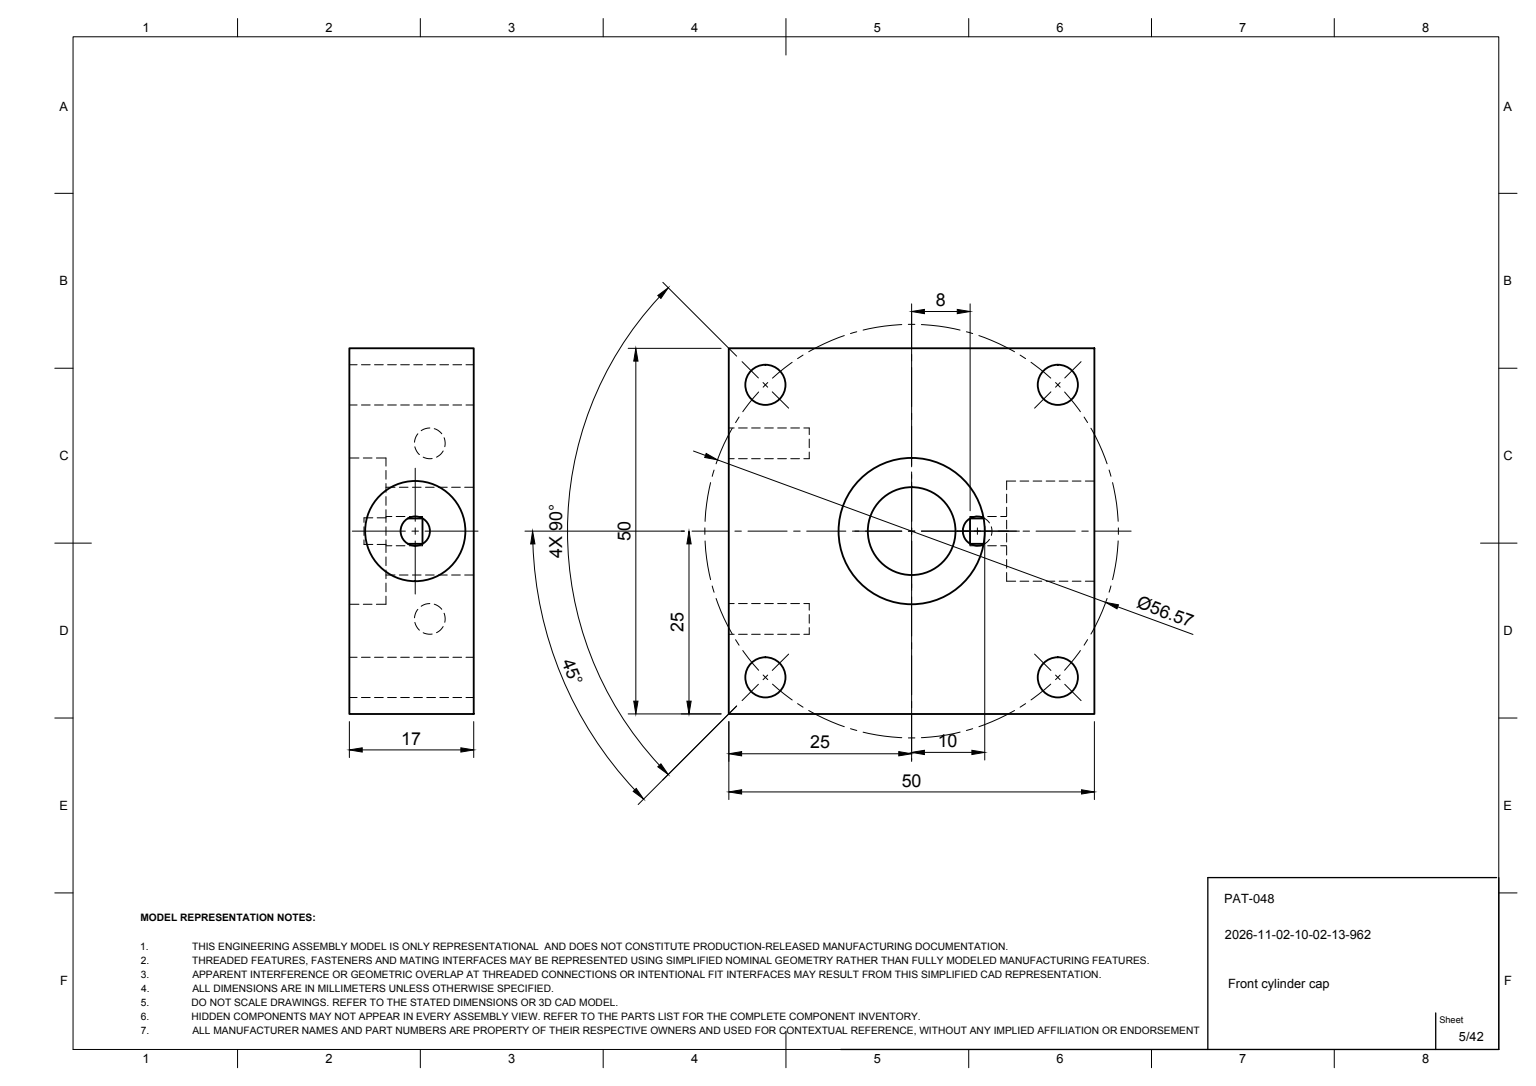
ISO-10303-21;
HEADER;
/* Generated by software containing ST-Developer
 * from STEP Tools, Inc. (www.steptools.com) 
 */

FILE_DESCRIPTION(
/* description */ ('Guided pneumatic stop gate'),
/* implementation_level */ '2;1');

FILE_NAME(
/* name */ 'Front cylinder cap.step',
/* time_stamp */ '2026-10-27T21:43:45-07:00',
/* author */ (''),
/* organization */ (''),
/* preprocessor_version */ 'ST-DEVELOPER v20.2',
/* originating_system */ 'Autodesk Translation Framework v15.17.0.0',
/* authorisation */ '');

FILE_SCHEMA (('AUTOMOTIVE_DESIGN { 1 0 10303 214 3 1 1 }'));
ENDSEC;

DATA;
#10=MECHANICAL_DESIGN_GEOMETRIC_PRESENTATION_REPRESENTATION('',(#535),#14392);
#451=SHAPE_REPRESENTATION_RELATIONSHIP('SRR','None',#14585,#493);
#493=ADVANCED_BREP_SHAPE_REPRESENTATION('',(#577),#14347);
#535=STYLED_ITEM('',(#14877),#577);
#577=MANIFOLD_SOLID_BREP('Body1',#7875);
#615=FACE_BOUND('',#1613,.T.);
#616=FACE_BOUND('',#1620,.T.);
#617=FACE_BOUND('',#1622,.T.);
#618=FACE_BOUND('',#1623,.T.);
#619=FACE_BOUND('',#1624,.T.);
#620=FACE_BOUND('',#1625,.T.);
#621=FACE_BOUND('',#1626,.T.);
#622=FACE_BOUND('',#1629,.T.);
#623=FACE_BOUND('',#1630,.T.);
#624=FACE_BOUND('',#1631,.T.);
#625=FACE_BOUND('',#1632,.T.);
#626=FACE_BOUND('',#1633,.T.);
#627=FACE_BOUND('',#1636,.T.);
#628=FACE_BOUND('',#1638,.T.);
#629=FACE_BOUND('',#1639,.T.);
#825=ELLIPSE('',#8400,0.282842712474619,0.2);
#826=ELLIPSE('',#8401,0.282842712474619,0.2);
#827=ELLIPSE('',#8403,0.282842712474619,0.2);
#828=ELLIPSE('',#8404,0.282842712474619,0.2);
#829=ELLIPSE('',#8408,0.282842712474619,0.2);
#830=ELLIPSE('',#8410,0.282842712474619,0.2);
#831=ELLIPSE('',#8412,0.282842712474619,0.2);
#839=PLANE('',#8390);
#840=PLANE('',#8394);
#841=PLANE('',#8395);
#842=PLANE('',#8397);
#843=PLANE('',#8413);
#844=PLANE('',#8415);
#845=PLANE('',#8416);
#846=PLANE('',#8418);
#847=PLANE('',#8429);
#848=PLANE('',#8433);
#849=PLANE('',#8449);
#850=PLANE('',#8450);
#851=PLANE('',#8451);
#852=PLANE('',#8452);
#853=PLANE('',#8453);
#854=PLANE('',#8454);
#855=PLANE('',#8455);
#1118=FACE_OUTER_BOUND('',#1593,.T.);
#1119=FACE_OUTER_BOUND('',#1594,.T.);
#1120=FACE_OUTER_BOUND('',#1595,.T.);
#1121=FACE_OUTER_BOUND('',#1596,.T.);
#1122=FACE_OUTER_BOUND('',#1597,.T.);
#1123=FACE_OUTER_BOUND('',#1598,.T.);
#1124=FACE_OUTER_BOUND('',#1599,.T.);
#1125=FACE_OUTER_BOUND('',#1600,.T.);
#1126=FACE_OUTER_BOUND('',#1601,.T.);
#1127=FACE_OUTER_BOUND('',#1602,.T.);
#1128=FACE_OUTER_BOUND('',#1603,.T.);
#1129=FACE_OUTER_BOUND('',#1604,.T.);
#1130=FACE_OUTER_BOUND('',#1605,.T.);
#1131=FACE_OUTER_BOUND('',#1606,.T.);
#1132=FACE_OUTER_BOUND('',#1607,.T.);
#1133=FACE_OUTER_BOUND('',#1608,.T.);
#1134=FACE_OUTER_BOUND('',#1609,.T.);
#1135=FACE_OUTER_BOUND('',#1610,.T.);
#1136=FACE_OUTER_BOUND('',#1611,.T.);
#1137=FACE_OUTER_BOUND('',#1612,.T.);
#1138=FACE_OUTER_BOUND('',#1614,.T.);
#1139=FACE_OUTER_BOUND('',#1615,.T.);
#1140=FACE_OUTER_BOUND('',#1616,.T.);
#1141=FACE_OUTER_BOUND('',#1617,.T.);
#1142=FACE_OUTER_BOUND('',#1618,.T.);
#1143=FACE_OUTER_BOUND('',#1619,.T.);
#1144=FACE_OUTER_BOUND('',#1621,.T.);
#1145=FACE_OUTER_BOUND('',#1627,.T.);
#1146=FACE_OUTER_BOUND('',#1628,.T.);
#1147=FACE_OUTER_BOUND('',#1634,.T.);
#1148=FACE_OUTER_BOUND('',#1635,.T.);
#1149=FACE_OUTER_BOUND('',#1637,.T.);
#1593=EDGE_LOOP('',(#5316,#5317,#5318,#5319));
#1594=EDGE_LOOP('',(#5320));
#1595=EDGE_LOOP('',(#5321,#5322,#5323,#5324));
#1596=EDGE_LOOP('',(#5325));
#1597=EDGE_LOOP('',(#5326,#5327));
#1598=EDGE_LOOP('',(#5328,#5329));
#1599=EDGE_LOOP('',(#5330,#5331,#5332));
#1600=EDGE_LOOP('',(#5333,#5334,#5335,#5336,#5337,#5338,#5339,#5340,#5341,
#5342,#5343,#5344,#5345));
#1601=EDGE_LOOP('',(#5346,#5347,#5348));
#1602=EDGE_LOOP('',(#5349,#5350));
#1603=EDGE_LOOP('',(#5351,#5352));
#1604=EDGE_LOOP('',(#5353,#5354));
#1605=EDGE_LOOP('',(#5355,#5356));
#1606=EDGE_LOOP('',(#5357,#5358,#5359));
#1607=EDGE_LOOP('',(#5360,#5361,#5362,#5363,#5364,#5365,#5366,#5367,#5368));
#1608=EDGE_LOOP('',(#5369,#5370,#5371));
#1609=EDGE_LOOP('',(#5372,#5373,#5374,#5375,#5376,#5377,#5378,#5379));
#1610=EDGE_LOOP('',(#5380,#5381));
#1611=EDGE_LOOP('',(#5382,#5383,#5384,#5385));
#1612=EDGE_LOOP('',(#5386));
#1613=EDGE_LOOP('',(#5387));
#1614=EDGE_LOOP('',(#5388,#5389,#5390,#5391));
#1615=EDGE_LOOP('',(#5392,#5393,#5394,#5395));
#1616=EDGE_LOOP('',(#5396,#5397,#5398,#5399));
#1617=EDGE_LOOP('',(#5400,#5401,#5402,#5403));
#1618=EDGE_LOOP('',(#5404,#5405,#5406,#5407));
#1619=EDGE_LOOP('',(#5408,#5409,#5410,#5411));
#1620=EDGE_LOOP('',(#5412));
#1621=EDGE_LOOP('',(#5413,#5414,#5415,#5416));
#1622=EDGE_LOOP('',(#5417));
#1623=EDGE_LOOP('',(#5418));
#1624=EDGE_LOOP('',(#5419));
#1625=EDGE_LOOP('',(#5420));
#1626=EDGE_LOOP('',(#5421));
#1627=EDGE_LOOP('',(#5422,#5423,#5424,#5425));
#1628=EDGE_LOOP('',(#5426,#5427,#5428,#5429));
#1629=EDGE_LOOP('',(#5430));
#1630=EDGE_LOOP('',(#5431));
#1631=EDGE_LOOP('',(#5432));
#1632=EDGE_LOOP('',(#5433));
#1633=EDGE_LOOP('',(#5434));
#1634=EDGE_LOOP('',(#5435,#5436,#5437,#5438));
#1635=EDGE_LOOP('',(#5439,#5440,#5441,#5442));
#1636=EDGE_LOOP('',(#5443));
#1637=EDGE_LOOP('',(#5444,#5445,#5446,#5447));
#1638=EDGE_LOOP('',(#5448));
#1639=EDGE_LOOP('',(#5449));
#2278=LINE('',#11927,#2823);
#2279=LINE('',#11934,#2824);
#2280=LINE('',#11940,#2825);
#2281=LINE('',#11944,#2826);
#2282=LINE('',#11952,#2827);
#2283=LINE('',#11954,#2828);
#2284=LINE('',#11959,#2829);
#2285=LINE('',#11963,#2830);
#2286=LINE('',#11967,#2831);
#2287=LINE('',#11978,#2832);
#2288=LINE('',#11986,#2833);
#2289=LINE('',#11994,#2834);
#2290=LINE('',#12002,#2835);
#2291=LINE('',#12009,#2836);
#2292=LINE('',#12015,#2837);
#2293=LINE('',#12021,#2838);
#2294=LINE('',#12027,#2839);
#2295=LINE('',#12033,#2840);
#2296=LINE('',#12039,#2841);
#2297=LINE('',#12041,#2842);
#2298=LINE('',#12043,#2843);
#2299=LINE('',#12044,#2844);
#2300=LINE('',#12047,#2845);
#2301=LINE('',#12049,#2846);
#2302=LINE('',#12050,#2847);
#2303=LINE('',#12053,#2848);
#2304=LINE('',#12055,#2849);
#2305=LINE('',#12056,#2850);
#2306=LINE('',#12058,#2851);
#2307=LINE('',#12059,#2852);
#2823=VECTOR('',#9391,0.21);
#2824=VECTOR('',#9400,0.21);
#2825=VECTOR('',#9407,1.);
#2826=VECTOR('',#9412,1.);
#2827=VECTOR('',#9423,1.);
#2828=VECTOR('',#9424,1.);
#2829=VECTOR('',#9429,0.2);
#2830=VECTOR('',#9432,1.);
#2831=VECTOR('',#9435,1.);
#2832=VECTOR('',#9454,1.);
#2833=VECTOR('',#9467,0.2);
#2834=VECTOR('',#9478,1.);
#2835=VECTOR('',#9489,0.685);
#2836=VECTOR('',#9498,0.275);
#2837=VECTOR('',#9505,0.275);
#2838=VECTOR('',#9512,0.275);
#2839=VECTOR('',#9519,0.275);
#2840=VECTOR('',#9526,0.6);
#2841=VECTOR('',#9533,1.);
#2842=VECTOR('',#9534,1.);
#2843=VECTOR('',#9535,1.);
#2844=VECTOR('',#9536,1.);
#2845=VECTOR('',#9539,1.);
#2846=VECTOR('',#9540,1.);
#2847=VECTOR('',#9541,1.);
#2848=VECTOR('',#9544,1.);
#2849=VECTOR('',#9545,1.);
#2850=VECTOR('',#9546,1.);
#2851=VECTOR('',#9549,1.);
#2852=VECTOR('',#9550,1.);
#3368=CIRCLE('',#8388,0.21);
#3369=CIRCLE('',#8389,0.21);
#3370=CIRCLE('',#8392,0.21);
#3371=CIRCLE('',#8393,0.21);
#3372=CIRCLE('',#8396,0.2);
#3373=CIRCLE('',#8398,0.2);
#3374=CIRCLE('',#8405,0.2);
#3375=CIRCLE('',#8406,0.2);
#3376=CIRCLE('',#8407,0.2);
#3377=CIRCLE('',#8411,0.2);
#3378=CIRCLE('',#8414,1.);
#3379=CIRCLE('',#8417,0.2);
#3380=CIRCLE('',#8419,0.2);
#3381=CIRCLE('',#8422,0.2);
#3382=CIRCLE('',#8424,0.2);
#3383=CIRCLE('',#8426,1.);
#3384=CIRCLE('',#8427,1.);
#3385=CIRCLE('',#8428,1.);
#3386=CIRCLE('',#8431,0.685);
#3387=CIRCLE('',#8432,0.685);
#3388=CIRCLE('',#8435,0.275);
#3389=CIRCLE('',#8436,0.275);
#3390=CIRCLE('',#8438,0.275);
#3391=CIRCLE('',#8439,0.275);
#3392=CIRCLE('',#8441,0.275);
#3393=CIRCLE('',#8442,0.275);
#3394=CIRCLE('',#8444,0.275);
#3395=CIRCLE('',#8445,0.275);
#3396=CIRCLE('',#8447,0.6);
#3397=CIRCLE('',#8448,0.6);
#3737=VERTEX_POINT('',#11924);
#3738=VERTEX_POINT('',#11926);
#3739=VERTEX_POINT('',#11931);
#3740=VERTEX_POINT('',#11933);
#3741=VERTEX_POINT('',#11938);
#3742=VERTEX_POINT('',#11939);
#3743=VERTEX_POINT('',#11943);
#3744=VERTEX_POINT('',#11947);
#3745=VERTEX_POINT('',#11951);
#3746=VERTEX_POINT('',#11953);
#3747=VERTEX_POINT('',#11956);
#3748=VERTEX_POINT('',#11958);
#3749=VERTEX_POINT('',#11960);
#3750=VERTEX_POINT('',#11962);
#3751=VERTEX_POINT('',#11964);
#3752=VERTEX_POINT('',#11966);
#3753=VERTEX_POINT('',#11971);
#3754=VERTEX_POINT('',#11985);
#3755=VERTEX_POINT('',#11991);
#3756=VERTEX_POINT('',#11993);
#3757=VERTEX_POINT('',#11999);
#3758=VERTEX_POINT('',#12001);
#3759=VERTEX_POINT('',#12006);
#3760=VERTEX_POINT('',#12008);
#3761=VERTEX_POINT('',#12012);
#3762=VERTEX_POINT('',#12014);
#3763=VERTEX_POINT('',#12018);
#3764=VERTEX_POINT('',#12020);
#3765=VERTEX_POINT('',#12024);
#3766=VERTEX_POINT('',#12026);
#3767=VERTEX_POINT('',#12030);
#3768=VERTEX_POINT('',#12032);
#3769=VERTEX_POINT('',#12037);
#3770=VERTEX_POINT('',#12038);
#3771=VERTEX_POINT('',#12040);
#3772=VERTEX_POINT('',#12042);
#3773=VERTEX_POINT('',#12046);
#3774=VERTEX_POINT('',#12048);
#3775=VERTEX_POINT('',#12052);
#3776=VERTEX_POINT('',#12054);
#4356=EDGE_CURVE('',#3737,#3737,#3368,.T.);
#4357=EDGE_CURVE('',#3737,#3738,#2278,.T.);
#4358=EDGE_CURVE('',#3738,#3738,#3369,.T.);
#4359=EDGE_CURVE('',#3739,#3739,#3370,.T.);
#4360=EDGE_CURVE('',#3739,#3740,#2279,.T.);
#4361=EDGE_CURVE('',#3740,#3740,#3371,.T.);
#4362=EDGE_CURVE('',#3741,#3742,#2280,.T.);
#4363=EDGE_CURVE('',#3741,#3742,#3372,.T.);
#4364=EDGE_CURVE('',#3743,#3741,#2281,.T.);
#4365=EDGE_CURVE('',#3743,#3741,#3373,.T.);
#4366=EDGE_CURVE('',#3744,#3743,#825,.T.);
#4367=EDGE_CURVE('',#3741,#3744,#826,.T.);
#4368=EDGE_CURVE('',#3742,#3745,#2282,.T.);
#4369=EDGE_CURVE('',#3746,#3741,#2283,.T.);
#4370=EDGE_CURVE('',#3744,#3746,#827,.T.);
#4371=EDGE_CURVE('',#3747,#3744,#828,.T.);
#4372=EDGE_CURVE('',#3747,#3748,#2284,.T.);
#4373=EDGE_CURVE('',#3749,#3748,#3374,.T.);
#4374=EDGE_CURVE('',#3750,#3749,#2285,.T.);
#4375=EDGE_CURVE('',#3750,#3751,#3375,.T.);
#4376=EDGE_CURVE('',#3752,#3751,#2286,.T.);
#4377=EDGE_CURVE('',#3748,#3752,#3376,.T.);
#4378=EDGE_CURVE('',#3745,#3747,#829,.T.);
#4379=EDGE_CURVE('',#3753,#3747,#830,.T.);
#4380=EDGE_CURVE('',#3742,#3753,#3377,.T.);
#4381=EDGE_CURVE('',#3747,#3742,#831,.T.);
#4382=EDGE_CURVE('',#3751,#3750,#3378,.T.);
#4383=EDGE_CURVE('',#3742,#3753,#2287,.T.);
#4384=EDGE_CURVE('',#3741,#3746,#3379,.T.);
#4385=EDGE_CURVE('',#3742,#3741,#3380,.T.);
#4386=EDGE_CURVE('',#3747,#3754,#2288,.T.);
#4387=EDGE_CURVE('',#3754,#3754,#3381,.T.);
#4388=EDGE_CURVE('',#3745,#3742,#3382,.T.);
#4389=EDGE_CURVE('',#3755,#3749,#3383,.T.);
#4390=EDGE_CURVE('',#3755,#3756,#2289,.T.);
#4391=EDGE_CURVE('',#3756,#3756,#3384,.T.);
#4392=EDGE_CURVE('',#3752,#3755,#3385,.T.);
#4393=EDGE_CURVE('',#3757,#3757,#3386,.T.);
#4394=EDGE_CURVE('',#3757,#3758,#2290,.T.);
#4395=EDGE_CURVE('',#3758,#3758,#3387,.T.);
#4396=EDGE_CURVE('',#3759,#3759,#3388,.T.);
#4397=EDGE_CURVE('',#3759,#3760,#2291,.T.);
#4398=EDGE_CURVE('',#3760,#3760,#3389,.T.);
#4399=EDGE_CURVE('',#3761,#3761,#3390,.T.);
#4400=EDGE_CURVE('',#3761,#3762,#2292,.T.);
#4401=EDGE_CURVE('',#3762,#3762,#3391,.T.);
#4402=EDGE_CURVE('',#3763,#3763,#3392,.T.);
#4403=EDGE_CURVE('',#3763,#3764,#2293,.T.);
#4404=EDGE_CURVE('',#3764,#3764,#3393,.T.);
#4405=EDGE_CURVE('',#3765,#3765,#3394,.T.);
#4406=EDGE_CURVE('',#3765,#3766,#2294,.T.);
#4407=EDGE_CURVE('',#3766,#3766,#3395,.T.);
#4408=EDGE_CURVE('',#3767,#3767,#3396,.T.);
#4409=EDGE_CURVE('',#3767,#3768,#2295,.T.);
#4410=EDGE_CURVE('',#3768,#3768,#3397,.T.);
#4411=EDGE_CURVE('',#3769,#3770,#2296,.T.);
#4412=EDGE_CURVE('',#3770,#3771,#2297,.T.);
#4413=EDGE_CURVE('',#3772,#3771,#2298,.T.);
#4414=EDGE_CURVE('',#3769,#3772,#2299,.T.);
#4415=EDGE_CURVE('',#3773,#3769,#2300,.T.);
#4416=EDGE_CURVE('',#3774,#3772,#2301,.T.);
#4417=EDGE_CURVE('',#3773,#3774,#2302,.T.);
#4418=EDGE_CURVE('',#3775,#3773,#2303,.T.);
#4419=EDGE_CURVE('',#3776,#3774,#2304,.T.);
#4420=EDGE_CURVE('',#3775,#3776,#2305,.T.);
#4421=EDGE_CURVE('',#3770,#3775,#2306,.T.);
#4422=EDGE_CURVE('',#3771,#3776,#2307,.T.);
#5316=ORIENTED_EDGE('',*,*,#4356,.F.);
#5317=ORIENTED_EDGE('',*,*,#4357,.T.);
#5318=ORIENTED_EDGE('',*,*,#4358,.T.);
#5319=ORIENTED_EDGE('',*,*,#4357,.F.);
#5320=ORIENTED_EDGE('',*,*,#4358,.F.);
#5321=ORIENTED_EDGE('',*,*,#4359,.F.);
#5322=ORIENTED_EDGE('',*,*,#4360,.T.);
#5323=ORIENTED_EDGE('',*,*,#4361,.T.);
#5324=ORIENTED_EDGE('',*,*,#4360,.F.);
#5325=ORIENTED_EDGE('',*,*,#4361,.F.);
#5326=ORIENTED_EDGE('',*,*,#4362,.F.);
#5327=ORIENTED_EDGE('',*,*,#4363,.T.);
#5328=ORIENTED_EDGE('',*,*,#4364,.F.);
#5329=ORIENTED_EDGE('',*,*,#4365,.T.);
#5330=ORIENTED_EDGE('',*,*,#4366,.F.);
#5331=ORIENTED_EDGE('',*,*,#4367,.F.);
#5332=ORIENTED_EDGE('',*,*,#4365,.F.);
#5333=ORIENTED_EDGE('',*,*,#4368,.F.);
#5334=ORIENTED_EDGE('',*,*,#4363,.F.);
#5335=ORIENTED_EDGE('',*,*,#4369,.F.);
#5336=ORIENTED_EDGE('',*,*,#4370,.F.);
#5337=ORIENTED_EDGE('',*,*,#4371,.F.);
#5338=ORIENTED_EDGE('',*,*,#4372,.T.);
#5339=ORIENTED_EDGE('',*,*,#4373,.F.);
#5340=ORIENTED_EDGE('',*,*,#4374,.F.);
#5341=ORIENTED_EDGE('',*,*,#4375,.T.);
#5342=ORIENTED_EDGE('',*,*,#4376,.F.);
#5343=ORIENTED_EDGE('',*,*,#4377,.F.);
#5344=ORIENTED_EDGE('',*,*,#4372,.F.);
#5345=ORIENTED_EDGE('',*,*,#4378,.F.);
#5346=ORIENTED_EDGE('',*,*,#4379,.F.);
#5347=ORIENTED_EDGE('',*,*,#4380,.F.);
#5348=ORIENTED_EDGE('',*,*,#4381,.F.);
#5349=ORIENTED_EDGE('',*,*,#4382,.F.);
#5350=ORIENTED_EDGE('',*,*,#4375,.F.);
#5351=ORIENTED_EDGE('',*,*,#4383,.F.);
#5352=ORIENTED_EDGE('',*,*,#4380,.T.);
#5353=ORIENTED_EDGE('',*,*,#4369,.T.);
#5354=ORIENTED_EDGE('',*,*,#4384,.T.);
#5355=ORIENTED_EDGE('',*,*,#4362,.T.);
#5356=ORIENTED_EDGE('',*,*,#4385,.T.);
#5357=ORIENTED_EDGE('',*,*,#4370,.T.);
#5358=ORIENTED_EDGE('',*,*,#4384,.F.);
#5359=ORIENTED_EDGE('',*,*,#4367,.T.);
#5360=ORIENTED_EDGE('',*,*,#4383,.T.);
#5361=ORIENTED_EDGE('',*,*,#4379,.T.);
#5362=ORIENTED_EDGE('',*,*,#4386,.T.);
#5363=ORIENTED_EDGE('',*,*,#4387,.F.);
#5364=ORIENTED_EDGE('',*,*,#4386,.F.);
#5365=ORIENTED_EDGE('',*,*,#4371,.T.);
#5366=ORIENTED_EDGE('',*,*,#4366,.T.);
#5367=ORIENTED_EDGE('',*,*,#4364,.T.);
#5368=ORIENTED_EDGE('',*,*,#4385,.F.);
#5369=ORIENTED_EDGE('',*,*,#4378,.T.);
#5370=ORIENTED_EDGE('',*,*,#4381,.T.);
#5371=ORIENTED_EDGE('',*,*,#4388,.F.);
#5372=ORIENTED_EDGE('',*,*,#4376,.T.);
#5373=ORIENTED_EDGE('',*,*,#4382,.T.);
#5374=ORIENTED_EDGE('',*,*,#4374,.T.);
#5375=ORIENTED_EDGE('',*,*,#4389,.F.);
#5376=ORIENTED_EDGE('',*,*,#4390,.T.);
#5377=ORIENTED_EDGE('',*,*,#4391,.F.);
#5378=ORIENTED_EDGE('',*,*,#4390,.F.);
#5379=ORIENTED_EDGE('',*,*,#4392,.F.);
#5380=ORIENTED_EDGE('',*,*,#4368,.T.);
#5381=ORIENTED_EDGE('',*,*,#4388,.T.);
#5382=ORIENTED_EDGE('',*,*,#4393,.F.);
#5383=ORIENTED_EDGE('',*,*,#4394,.T.);
#5384=ORIENTED_EDGE('',*,*,#4395,.F.);
#5385=ORIENTED_EDGE('',*,*,#4394,.F.);
#5386=ORIENTED_EDGE('',*,*,#4393,.T.);
#5387=ORIENTED_EDGE('',*,*,#4387,.T.);
#5388=ORIENTED_EDGE('',*,*,#4396,.F.);
#5389=ORIENTED_EDGE('',*,*,#4397,.T.);
#5390=ORIENTED_EDGE('',*,*,#4398,.F.);
#5391=ORIENTED_EDGE('',*,*,#4397,.F.);
#5392=ORIENTED_EDGE('',*,*,#4399,.F.);
#5393=ORIENTED_EDGE('',*,*,#4400,.T.);
#5394=ORIENTED_EDGE('',*,*,#4401,.F.);
#5395=ORIENTED_EDGE('',*,*,#4400,.F.);
#5396=ORIENTED_EDGE('',*,*,#4402,.F.);
#5397=ORIENTED_EDGE('',*,*,#4403,.T.);
#5398=ORIENTED_EDGE('',*,*,#4404,.F.);
#5399=ORIENTED_EDGE('',*,*,#4403,.F.);
#5400=ORIENTED_EDGE('',*,*,#4405,.F.);
#5401=ORIENTED_EDGE('',*,*,#4406,.T.);
#5402=ORIENTED_EDGE('',*,*,#4407,.F.);
#5403=ORIENTED_EDGE('',*,*,#4406,.F.);
#5404=ORIENTED_EDGE('',*,*,#4408,.F.);
#5405=ORIENTED_EDGE('',*,*,#4409,.T.);
#5406=ORIENTED_EDGE('',*,*,#4410,.F.);
#5407=ORIENTED_EDGE('',*,*,#4409,.F.);
#5408=ORIENTED_EDGE('',*,*,#4373,.T.);
#5409=ORIENTED_EDGE('',*,*,#4377,.T.);
#5410=ORIENTED_EDGE('',*,*,#4392,.T.);
#5411=ORIENTED_EDGE('',*,*,#4389,.T.);
#5412=ORIENTED_EDGE('',*,*,#4410,.T.);
#5413=ORIENTED_EDGE('',*,*,#4411,.T.);
#5414=ORIENTED_EDGE('',*,*,#4412,.T.);
#5415=ORIENTED_EDGE('',*,*,#4413,.F.);
#5416=ORIENTED_EDGE('',*,*,#4414,.F.);
#5417=ORIENTED_EDGE('',*,*,#4391,.T.);
#5418=ORIENTED_EDGE('',*,*,#4407,.T.);
#5419=ORIENTED_EDGE('',*,*,#4404,.T.);
#5420=ORIENTED_EDGE('',*,*,#4401,.T.);
#5421=ORIENTED_EDGE('',*,*,#4398,.T.);
#5422=ORIENTED_EDGE('',*,*,#4415,.T.);
#5423=ORIENTED_EDGE('',*,*,#4414,.T.);
#5424=ORIENTED_EDGE('',*,*,#4416,.F.);
#5425=ORIENTED_EDGE('',*,*,#4417,.F.);
#5426=ORIENTED_EDGE('',*,*,#4418,.T.);
#5427=ORIENTED_EDGE('',*,*,#4417,.T.);
#5428=ORIENTED_EDGE('',*,*,#4419,.F.);
#5429=ORIENTED_EDGE('',*,*,#4420,.F.);
#5430=ORIENTED_EDGE('',*,*,#4408,.T.);
#5431=ORIENTED_EDGE('',*,*,#4405,.T.);
#5432=ORIENTED_EDGE('',*,*,#4402,.T.);
#5433=ORIENTED_EDGE('',*,*,#4399,.T.);
#5434=ORIENTED_EDGE('',*,*,#4396,.T.);
#5435=ORIENTED_EDGE('',*,*,#4421,.T.);
#5436=ORIENTED_EDGE('',*,*,#4420,.T.);
#5437=ORIENTED_EDGE('',*,*,#4422,.F.);
#5438=ORIENTED_EDGE('',*,*,#4412,.F.);
#5439=ORIENTED_EDGE('',*,*,#4422,.T.);
#5440=ORIENTED_EDGE('',*,*,#4419,.T.);
#5441=ORIENTED_EDGE('',*,*,#4416,.T.);
#5442=ORIENTED_EDGE('',*,*,#4413,.T.);
#5443=ORIENTED_EDGE('',*,*,#4395,.T.);
#5444=ORIENTED_EDGE('',*,*,#4421,.F.);
#5445=ORIENTED_EDGE('',*,*,#4411,.F.);
#5446=ORIENTED_EDGE('',*,*,#4415,.F.);
#5447=ORIENTED_EDGE('',*,*,#4418,.F.);
#5448=ORIENTED_EDGE('',*,*,#4356,.T.);
#5449=ORIENTED_EDGE('',*,*,#4359,.T.);
#7236=CYLINDRICAL_SURFACE('',#8387,0.21);
#7237=CYLINDRICAL_SURFACE('',#8391,0.21);
#7238=CYLINDRICAL_SURFACE('',#8399,0.2);
#7239=CYLINDRICAL_SURFACE('',#8402,0.2);
#7240=CYLINDRICAL_SURFACE('',#8409,0.2);
#7241=CYLINDRICAL_SURFACE('',#8420,0.2);
#7242=CYLINDRICAL_SURFACE('',#8421,0.2);
#7243=CYLINDRICAL_SURFACE('',#8423,0.2);
#7244=CYLINDRICAL_SURFACE('',#8425,1.);
#7245=CYLINDRICAL_SURFACE('',#8430,0.685);
#7246=CYLINDRICAL_SURFACE('',#8434,0.275);
#7247=CYLINDRICAL_SURFACE('',#8437,0.275);
#7248=CYLINDRICAL_SURFACE('',#8440,0.275);
#7249=CYLINDRICAL_SURFACE('',#8443,0.275);
#7250=CYLINDRICAL_SURFACE('',#8446,0.6);
#7400=ADVANCED_FACE('',(#1118),#7236,.F.);
#7401=ADVANCED_FACE('',(#1119),#839,.F.);
#7402=ADVANCED_FACE('',(#1120),#7237,.F.);
#7403=ADVANCED_FACE('',(#1121),#840,.F.);
#7404=ADVANCED_FACE('',(#1122),#841,.T.);
#7405=ADVANCED_FACE('',(#1123),#842,.T.);
#7406=ADVANCED_FACE('',(#1124),#7238,.F.);
#7407=ADVANCED_FACE('',(#1125),#7239,.F.);
#7408=ADVANCED_FACE('',(#1126),#7240,.F.);
#7409=ADVANCED_FACE('',(#1127),#843,.F.);
#7410=ADVANCED_FACE('',(#1128),#844,.T.);
#7411=ADVANCED_FACE('',(#1129),#845,.T.);
#7412=ADVANCED_FACE('',(#1130),#846,.T.);
#7413=ADVANCED_FACE('',(#1131),#7241,.F.);
#7414=ADVANCED_FACE('',(#1132),#7242,.F.);
#7415=ADVANCED_FACE('',(#1133),#7243,.F.);
#7416=ADVANCED_FACE('',(#1134),#7244,.F.);
#7417=ADVANCED_FACE('',(#1135),#847,.T.);
#7418=ADVANCED_FACE('',(#1136),#7245,.F.);
#7419=ADVANCED_FACE('',(#1137,#615),#848,.T.);
#7420=ADVANCED_FACE('',(#1138),#7246,.F.);
#7421=ADVANCED_FACE('',(#1139),#7247,.F.);
#7422=ADVANCED_FACE('',(#1140),#7248,.F.);
#7423=ADVANCED_FACE('',(#1141),#7249,.F.);
#7424=ADVANCED_FACE('',(#1142),#7250,.F.);
#7425=ADVANCED_FACE('',(#1143,#616),#849,.T.);
#7426=ADVANCED_FACE('',(#1144,#617,#618,#619,#620,#621),#850,.T.);
#7427=ADVANCED_FACE('',(#1145),#851,.T.);
#7428=ADVANCED_FACE('',(#1146,#622,#623,#624,#625,#626),#852,.T.);
#7429=ADVANCED_FACE('',(#1147),#853,.T.);
#7430=ADVANCED_FACE('',(#1148,#627),#854,.T.);
#7431=ADVANCED_FACE('',(#1149,#628,#629),#855,.F.);
#7875=CLOSED_SHELL('',(#7400,#7401,#7402,#7403,#7404,#7405,#7406,#7407,
#7408,#7409,#7410,#7411,#7412,#7413,#7414,#7415,#7416,#7417,#7418,#7419,
#7420,#7421,#7422,#7423,#7424,#7425,#7426,#7427,#7428,#7429,#7430,#7431));
#8386=AXIS2_PLACEMENT_3D('',#11922,#9385,#9386);
#8387=AXIS2_PLACEMENT_3D('',#11923,#9387,#9388);
#8388=AXIS2_PLACEMENT_3D('',#11925,#9389,#9390);
#8389=AXIS2_PLACEMENT_3D('',#11928,#9392,#9393);
#8390=AXIS2_PLACEMENT_3D('',#11929,#9394,#9395);
#8391=AXIS2_PLACEMENT_3D('',#11930,#9396,#9397);
#8392=AXIS2_PLACEMENT_3D('',#11932,#9398,#9399);
#8393=AXIS2_PLACEMENT_3D('',#11935,#9401,#9402);
#8394=AXIS2_PLACEMENT_3D('',#11936,#9403,#9404);
#8395=AXIS2_PLACEMENT_3D('',#11937,#9405,#9406);
#8396=AXIS2_PLACEMENT_3D('',#11941,#9408,#9409);
#8397=AXIS2_PLACEMENT_3D('',#11942,#9410,#9411);
#8398=AXIS2_PLACEMENT_3D('',#11945,#9413,#9414);
#8399=AXIS2_PLACEMENT_3D('',#11946,#9415,#9416);
#8400=AXIS2_PLACEMENT_3D('',#11948,#9417,#9418);
#8401=AXIS2_PLACEMENT_3D('',#11949,#9419,#9420);
#8402=AXIS2_PLACEMENT_3D('',#11950,#9421,#9422);
#8403=AXIS2_PLACEMENT_3D('',#11955,#9425,#9426);
#8404=AXIS2_PLACEMENT_3D('',#11957,#9427,#9428);
#8405=AXIS2_PLACEMENT_3D('',#11961,#9430,#9431);
#8406=AXIS2_PLACEMENT_3D('',#11965,#9433,#9434);
#8407=AXIS2_PLACEMENT_3D('',#11968,#9436,#9437);
#8408=AXIS2_PLACEMENT_3D('',#11969,#9438,#9439);
#8409=AXIS2_PLACEMENT_3D('',#11970,#9440,#9441);
#8410=AXIS2_PLACEMENT_3D('',#11972,#9442,#9443);
#8411=AXIS2_PLACEMENT_3D('',#11973,#9444,#9445);
#8412=AXIS2_PLACEMENT_3D('',#11974,#9446,#9447);
#8413=AXIS2_PLACEMENT_3D('',#11975,#9448,#9449);
#8414=AXIS2_PLACEMENT_3D('',#11976,#9450,#9451);
#8415=AXIS2_PLACEMENT_3D('',#11977,#9452,#9453);
#8416=AXIS2_PLACEMENT_3D('',#11979,#9455,#9456);
#8417=AXIS2_PLACEMENT_3D('',#11980,#9457,#9458);
#8418=AXIS2_PLACEMENT_3D('',#11981,#9459,#9460);
#8419=AXIS2_PLACEMENT_3D('',#11982,#9461,#9462);
#8420=AXIS2_PLACEMENT_3D('',#11983,#9463,#9464);
#8421=AXIS2_PLACEMENT_3D('',#11984,#9465,#9466);
#8422=AXIS2_PLACEMENT_3D('',#11987,#9468,#9469);
#8423=AXIS2_PLACEMENT_3D('',#11988,#9470,#9471);
#8424=AXIS2_PLACEMENT_3D('',#11989,#9472,#9473);
#8425=AXIS2_PLACEMENT_3D('',#11990,#9474,#9475);
#8426=AXIS2_PLACEMENT_3D('',#11992,#9476,#9477);
#8427=AXIS2_PLACEMENT_3D('',#11995,#9479,#9480);
#8428=AXIS2_PLACEMENT_3D('',#11996,#9481,#9482);
#8429=AXIS2_PLACEMENT_3D('',#11997,#9483,#9484);
#8430=AXIS2_PLACEMENT_3D('',#11998,#9485,#9486);
#8431=AXIS2_PLACEMENT_3D('',#12000,#9487,#9488);
#8432=AXIS2_PLACEMENT_3D('',#12003,#9490,#9491);
#8433=AXIS2_PLACEMENT_3D('',#12004,#9492,#9493);
#8434=AXIS2_PLACEMENT_3D('',#12005,#9494,#9495);
#8435=AXIS2_PLACEMENT_3D('',#12007,#9496,#9497);
#8436=AXIS2_PLACEMENT_3D('',#12010,#9499,#9500);
#8437=AXIS2_PLACEMENT_3D('',#12011,#9501,#9502);
#8438=AXIS2_PLACEMENT_3D('',#12013,#9503,#9504);
#8439=AXIS2_PLACEMENT_3D('',#12016,#9506,#9507);
#8440=AXIS2_PLACEMENT_3D('',#12017,#9508,#9509);
#8441=AXIS2_PLACEMENT_3D('',#12019,#9510,#9511);
#8442=AXIS2_PLACEMENT_3D('',#12022,#9513,#9514);
#8443=AXIS2_PLACEMENT_3D('',#12023,#9515,#9516);
#8444=AXIS2_PLACEMENT_3D('',#12025,#9517,#9518);
#8445=AXIS2_PLACEMENT_3D('',#12028,#9520,#9521);
#8446=AXIS2_PLACEMENT_3D('',#12029,#9522,#9523);
#8447=AXIS2_PLACEMENT_3D('',#12031,#9524,#9525);
#8448=AXIS2_PLACEMENT_3D('',#12034,#9527,#9528);
#8449=AXIS2_PLACEMENT_3D('',#12035,#9529,#9530);
#8450=AXIS2_PLACEMENT_3D('',#12036,#9531,#9532);
#8451=AXIS2_PLACEMENT_3D('',#12045,#9537,#9538);
#8452=AXIS2_PLACEMENT_3D('',#12051,#9542,#9543);
#8453=AXIS2_PLACEMENT_3D('',#12057,#9547,#9548);
#8454=AXIS2_PLACEMENT_3D('',#12060,#9551,#9552);
#8455=AXIS2_PLACEMENT_3D('',#12061,#9553,#9554);
#9385=DIRECTION('axis',(0.,0.,1.));
#9386=DIRECTION('refdir',(1.,0.,0.));
#9387=DIRECTION('center_axis',(0.,0.,1.));
#9388=DIRECTION('ref_axis',(1.,0.,0.));
#9389=DIRECTION('center_axis',(0.,0.,1.));
#9390=DIRECTION('ref_axis',(1.,0.,0.));
#9391=DIRECTION('',(0.,0.,1.));
#9392=DIRECTION('center_axis',(0.,0.,1.));
#9393=DIRECTION('ref_axis',(1.,0.,0.));
#9394=DIRECTION('center_axis',(0.,0.,1.));
#9395=DIRECTION('ref_axis',(1.,0.,0.));
#9396=DIRECTION('center_axis',(0.,0.,1.));
#9397=DIRECTION('ref_axis',(1.,0.,0.));
#9398=DIRECTION('center_axis',(0.,0.,1.));
#9399=DIRECTION('ref_axis',(1.,0.,0.));
#9400=DIRECTION('',(0.,0.,1.));
#9401=DIRECTION('center_axis',(0.,0.,1.));
#9402=DIRECTION('ref_axis',(1.,0.,0.));
#9403=DIRECTION('center_axis',(0.,0.,1.));
#9404=DIRECTION('ref_axis',(1.,0.,0.));
#9405=DIRECTION('center_axis',(0.,1.,0.));
#9406=DIRECTION('ref_axis',(1.,0.,0.));
#9407=DIRECTION('',(-1.,0.,0.));
#9408=DIRECTION('center_axis',(0.,1.,0.));
#9409=DIRECTION('ref_axis',(1.,0.,0.));
#9410=DIRECTION('center_axis',(0.,1.,0.));
#9411=DIRECTION('ref_axis',(1.,0.,0.));
#9412=DIRECTION('',(0.,0.,-1.));
#9413=DIRECTION('center_axis',(0.,1.,0.));
#9414=DIRECTION('ref_axis',(1.,0.,0.));
#9415=DIRECTION('center_axis',(0.,1.,0.));
#9416=DIRECTION('ref_axis',(1.,0.,0.));
#9417=DIRECTION('center_axis',(0.,-0.707106781186548,-0.707106781186547));
#9418=DIRECTION('ref_axis',(0.,0.707106781186547,-0.707106781186548));
#9419=DIRECTION('center_axis',(0.,-0.707106781186548,0.707106781186547));
#9420=DIRECTION('ref_axis',(0.,-0.707106781186547,-0.707106781186548));
#9421=DIRECTION('center_axis',(0.,1.,0.));
#9422=DIRECTION('ref_axis',(1.,0.,0.));
#9423=DIRECTION('',(0.,1.,0.));
#9424=DIRECTION('',(0.,-1.,0.));
#9425=DIRECTION('center_axis',(0.,0.707106781186548,0.707106781186547));
#9426=DIRECTION('ref_axis',(0.,0.707106781186547,-0.707106781186548));
#9427=DIRECTION('center_axis',(0.,0.707106781186548,-0.707106781186547));
#9428=DIRECTION('ref_axis',(0.,-0.707106781186547,-0.707106781186548));
#9429=DIRECTION('',(0.,1.,0.));
#9430=DIRECTION('center_axis',(0.,-1.,0.));
#9431=DIRECTION('ref_axis',(1.,0.,0.));
#9432=DIRECTION('',(0.,-1.,0.));
#9433=DIRECTION('center_axis',(0.,1.,0.));
#9434=DIRECTION('ref_axis',(1.,0.,0.));
#9435=DIRECTION('',(0.,1.,0.));
#9436=DIRECTION('center_axis',(0.,-1.,0.));
#9437=DIRECTION('ref_axis',(1.,0.,0.));
#9438=DIRECTION('center_axis',(0.,0.707106781186548,0.707106781186547));
#9439=DIRECTION('ref_axis',(0.,0.707106781186547,-0.707106781186548));
#9440=DIRECTION('center_axis',(0.,1.,0.));
#9441=DIRECTION('ref_axis',(-1.,0.,-2.54207057918564E-15));
#9442=DIRECTION('center_axis',(0.,-0.707106781186548,-0.707106781186547));
#9443=DIRECTION('ref_axis',(0.,0.707106781186547,-0.707106781186548));
#9444=DIRECTION('center_axis',(0.,1.,0.));
#9445=DIRECTION('ref_axis',(1.,0.,0.));
#9446=DIRECTION('center_axis',(0.,-0.707106781186548,0.707106781186547));
#9447=DIRECTION('ref_axis',(0.,-0.707106781186547,-0.707106781186548));
#9448=DIRECTION('center_axis',(0.,1.,0.));
#9449=DIRECTION('ref_axis',(1.,0.,0.));
#9450=DIRECTION('center_axis',(0.,-1.,0.));
#9451=DIRECTION('ref_axis',(1.,0.,0.));
#9452=DIRECTION('center_axis',(0.,1.,0.));
#9453=DIRECTION('ref_axis',(1.,0.,0.));
#9454=DIRECTION('',(0.,0.,1.));
#9455=DIRECTION('center_axis',(0.,0.,1.));
#9456=DIRECTION('ref_axis',(1.,0.,0.));
#9457=DIRECTION('center_axis',(0.,0.,1.));
#9458=DIRECTION('ref_axis',(1.,0.,0.));
#9459=DIRECTION('center_axis',(0.,0.,1.));
#9460=DIRECTION('ref_axis',(1.,0.,0.));
#9461=DIRECTION('center_axis',(0.,0.,1.));
#9462=DIRECTION('ref_axis',(1.,0.,0.));
#9463=DIRECTION('center_axis',(0.,0.,1.));
#9464=DIRECTION('ref_axis',(1.,0.,0.));
#9465=DIRECTION('center_axis',(0.,0.,1.));
#9466=DIRECTION('ref_axis',(1.,0.,0.));
#9467=DIRECTION('',(0.,0.,1.));
#9468=DIRECTION('center_axis',(0.,0.,-1.));
#9469=DIRECTION('ref_axis',(1.,0.,0.));
#9470=DIRECTION('center_axis',(0.,0.,1.));
#9471=DIRECTION('ref_axis',(-1.,-1.65389215948552E-15,0.));
#9472=DIRECTION('center_axis',(0.,0.,1.));
#9473=DIRECTION('ref_axis',(1.,0.,0.));
#9474=DIRECTION('center_axis',(0.,1.,0.));
#9475=DIRECTION('ref_axis',(1.,0.,0.));
#9476=DIRECTION('center_axis',(0.,1.,0.));
#9477=DIRECTION('ref_axis',(1.,0.,0.));
#9478=DIRECTION('',(0.,1.,0.));
#9479=DIRECTION('center_axis',(0.,-1.,0.));
#9480=DIRECTION('ref_axis',(1.,0.,0.));
#9481=DIRECTION('center_axis',(0.,1.,0.));
#9482=DIRECTION('ref_axis',(1.,0.,0.));
#9483=DIRECTION('center_axis',(0.,0.,1.));
#9484=DIRECTION('ref_axis',(1.,0.,0.));
#9485=DIRECTION('center_axis',(0.,0.,1.));
#9486=DIRECTION('ref_axis',(1.,0.,0.));
#9487=DIRECTION('center_axis',(0.,0.,1.));
#9488=DIRECTION('ref_axis',(1.,0.,0.));
#9489=DIRECTION('',(0.,0.,1.));
#9490=DIRECTION('center_axis',(0.,0.,-1.));
#9491=DIRECTION('ref_axis',(1.,0.,0.));
#9492=DIRECTION('center_axis',(0.,0.,1.));
#9493=DIRECTION('ref_axis',(1.,0.,0.));
#9494=DIRECTION('center_axis',(0.,1.,0.));
#9495=DIRECTION('ref_axis',(1.,0.,0.));
#9496=DIRECTION('center_axis',(0.,1.,0.));
#9497=DIRECTION('ref_axis',(1.,0.,0.));
#9498=DIRECTION('',(0.,1.,0.));
#9499=DIRECTION('center_axis',(0.,-1.,0.));
#9500=DIRECTION('ref_axis',(1.,0.,0.));
#9501=DIRECTION('center_axis',(0.,1.,0.));
#9502=DIRECTION('ref_axis',(1.,0.,0.));
#9503=DIRECTION('center_axis',(0.,1.,0.));
#9504=DIRECTION('ref_axis',(1.,0.,0.));
#9505=DIRECTION('',(0.,1.,0.));
#9506=DIRECTION('center_axis',(0.,-1.,0.));
#9507=DIRECTION('ref_axis',(1.,0.,0.));
#9508=DIRECTION('center_axis',(0.,1.,0.));
#9509=DIRECTION('ref_axis',(1.,0.,0.));
#9510=DIRECTION('center_axis',(0.,1.,0.));
#9511=DIRECTION('ref_axis',(1.,0.,0.));
#9512=DIRECTION('',(0.,1.,0.));
#9513=DIRECTION('center_axis',(0.,-1.,0.));
#9514=DIRECTION('ref_axis',(1.,0.,0.));
#9515=DIRECTION('center_axis',(0.,1.,0.));
#9516=DIRECTION('ref_axis',(1.,0.,0.));
#9517=DIRECTION('center_axis',(0.,1.,0.));
#9518=DIRECTION('ref_axis',(1.,0.,0.));
#9519=DIRECTION('',(0.,1.,0.));
#9520=DIRECTION('center_axis',(0.,-1.,0.));
#9521=DIRECTION('ref_axis',(1.,0.,0.));
#9522=DIRECTION('center_axis',(0.,1.,0.));
#9523=DIRECTION('ref_axis',(1.,0.,0.));
#9524=DIRECTION('center_axis',(0.,1.,0.));
#9525=DIRECTION('ref_axis',(1.,0.,0.));
#9526=DIRECTION('',(0.,1.,0.));
#9527=DIRECTION('center_axis',(0.,-1.,0.));
#9528=DIRECTION('ref_axis',(1.,0.,0.));
#9529=DIRECTION('center_axis',(0.,1.,0.));
#9530=DIRECTION('ref_axis',(1.,0.,0.));
#9531=DIRECTION('center_axis',(0.,1.,0.));
#9532=DIRECTION('ref_axis',(-1.,0.,0.));
#9533=DIRECTION('',(-1.,0.,0.));
#9534=DIRECTION('',(0.,0.,1.));
#9535=DIRECTION('',(-1.,0.,0.));
#9536=DIRECTION('',(0.,0.,1.));
#9537=DIRECTION('center_axis',(1.,0.,0.));
#9538=DIRECTION('ref_axis',(0.,1.,0.));
#9539=DIRECTION('',(0.,1.,0.));
#9540=DIRECTION('',(0.,1.,0.));
#9541=DIRECTION('',(0.,0.,1.));
#9542=DIRECTION('center_axis',(0.,-1.,0.));
#9543=DIRECTION('ref_axis',(1.,0.,0.));
#9544=DIRECTION('',(1.,0.,0.));
#9545=DIRECTION('',(1.,0.,0.));
#9546=DIRECTION('',(0.,0.,1.));
#9547=DIRECTION('center_axis',(-1.,0.,0.));
#9548=DIRECTION('ref_axis',(0.,-1.,0.));
#9549=DIRECTION('',(0.,-1.,0.));
#9550=DIRECTION('',(0.,-1.,0.));
#9551=DIRECTION('center_axis',(0.,0.,1.));
#9552=DIRECTION('ref_axis',(1.,0.,0.));
#9553=DIRECTION('center_axis',(0.,0.,1.));
#9554=DIRECTION('ref_axis',(1.,0.,0.));
#11922=CARTESIAN_POINT('',(0.,0.,0.));
#11923=CARTESIAN_POINT('Origin',(-1.2,0.6,1.9));
#11924=CARTESIAN_POINT('',(-1.41,0.6,2.));
#11925=CARTESIAN_POINT('Origin',(-1.2,0.6,2.));
#11926=CARTESIAN_POINT('',(-1.41,0.6,3.1));
#11927=CARTESIAN_POINT('',(-1.41,0.6,1.9));
#11928=CARTESIAN_POINT('Origin',(-1.2,0.6,3.1));
#11929=CARTESIAN_POINT('Origin',(-1.2,0.6,3.1));
#11930=CARTESIAN_POINT('Origin',(1.2,0.6,1.9));
#11931=CARTESIAN_POINT('',(0.99,0.6,2.));
#11932=CARTESIAN_POINT('Origin',(1.2,0.6,2.));
#11933=CARTESIAN_POINT('',(0.99,0.6,3.1));
#11934=CARTESIAN_POINT('',(0.99,0.6,1.9));
#11935=CARTESIAN_POINT('Origin',(1.2,0.6,3.1));
#11936=CARTESIAN_POINT('Origin',(1.2,0.6,3.1));
#11937=CARTESIAN_POINT('Origin',(0.,0.7,5.4));
#11938=CARTESIAN_POINT('',(0.173205080756888,0.7,5.3));
#11939=CARTESIAN_POINT('',(-0.173205080756888,0.7,5.3));
#11940=CARTESIAN_POINT('',(0.,0.7,5.3));
#11941=CARTESIAN_POINT('Origin',(0.,0.7,5.4));
#11942=CARTESIAN_POINT('Origin',(0.,0.7,5.4));
#11943=CARTESIAN_POINT('',(0.173205080756888,0.7,5.5));
#11944=CARTESIAN_POINT('',(0.173205080756888,0.7,5.3));
#11945=CARTESIAN_POINT('Origin',(0.,0.7,5.4));
#11946=CARTESIAN_POINT('Origin',(0.,0.7,5.4));
#11947=CARTESIAN_POINT('',(0.2,0.8,5.4));
#11948=CARTESIAN_POINT('Origin',(0.,0.8,5.4));
#11949=CARTESIAN_POINT('Origin',(0.,0.8,5.4));
#11950=CARTESIAN_POINT('Origin',(0.,0.7,5.4));
#11951=CARTESIAN_POINT('',(-0.173205080756888,0.9,5.3));
#11952=CARTESIAN_POINT('',(-0.173205080756888,0.7,5.3));
#11953=CARTESIAN_POINT('',(0.173205080756888,0.9,5.3));
#11954=CARTESIAN_POINT('',(0.173205080756888,0.7,5.3));
#11955=CARTESIAN_POINT('Origin',(0.,0.8,5.4));
#11956=CARTESIAN_POINT('',(-0.2,0.8,5.4));
#11957=CARTESIAN_POINT('Origin',(0.,0.8,5.4));
#11958=CARTESIAN_POINT('',(-0.2,1.2,5.4));
#11959=CARTESIAN_POINT('',(-0.2,0.7,5.4));
#11960=CARTESIAN_POINT('',(-0.181811868577262,1.2,5.48333333333333));
#11961=CARTESIAN_POINT('Origin',(0.,1.2,5.4));
#11962=CARTESIAN_POINT('',(-0.181811868577262,1.5,5.48333333333333));
#11963=CARTESIAN_POINT('',(-0.181811868577262,0.7,5.48333333333333));
#11964=CARTESIAN_POINT('',(0.181811868577262,1.5,5.48333333333333));
#11965=CARTESIAN_POINT('Origin',(0.,1.5,5.4));
#11966=CARTESIAN_POINT('',(0.181811868577262,1.2,5.48333333333333));
#11967=CARTESIAN_POINT('',(0.181811868577262,0.7,5.48333333333333));
#11968=CARTESIAN_POINT('Origin',(0.,1.2,5.4));
#11969=CARTESIAN_POINT('Origin',(0.,0.8,5.4));
#11970=CARTESIAN_POINT('Origin',(0.,0.7,5.4));
#11971=CARTESIAN_POINT('',(-0.173205080756888,0.7,5.5));
#11972=CARTESIAN_POINT('Origin',(0.,0.8,5.4));
#11973=CARTESIAN_POINT('Origin',(0.,0.7,5.4));
#11974=CARTESIAN_POINT('Origin',(0.,0.8,5.4));
#11975=CARTESIAN_POINT('Origin',(0.,1.5,5.4));
#11976=CARTESIAN_POINT('Origin',(0.,1.5,4.5));
#11977=CARTESIAN_POINT('Origin',(0.,0.7,5.4));
#11978=CARTESIAN_POINT('',(-0.173205080756888,0.7,5.3));
#11979=CARTESIAN_POINT('Origin',(0.,0.8,5.3));
#11980=CARTESIAN_POINT('Origin',(0.,0.8,5.3));
#11981=CARTESIAN_POINT('Origin',(0.,0.8,5.3));
#11982=CARTESIAN_POINT('Origin',(0.,0.8,5.3));
#11983=CARTESIAN_POINT('Origin',(0.,0.8,5.3));
#11984=CARTESIAN_POINT('Origin',(0.,0.8,5.3));
#11985=CARTESIAN_POINT('',(-0.2,0.8,5.8));
#11986=CARTESIAN_POINT('',(-0.2,0.8,5.3));
#11987=CARTESIAN_POINT('Origin',(0.,0.8,5.8));
#11988=CARTESIAN_POINT('Origin',(0.,0.8,5.3));
#11989=CARTESIAN_POINT('Origin',(0.,0.8,5.3));
#11990=CARTESIAN_POINT('Origin',(0.,1.2,4.5));
#11991=CARTESIAN_POINT('',(-1.,1.2,4.5));
#11992=CARTESIAN_POINT('Origin',(0.,1.2,4.5));
#11993=CARTESIAN_POINT('',(-1.,1.7,4.5));
#11994=CARTESIAN_POINT('',(-1.,1.2,4.5));
#11995=CARTESIAN_POINT('Origin',(0.,1.7,4.5));
#11996=CARTESIAN_POINT('Origin',(0.,1.2,4.5));
#11997=CARTESIAN_POINT('Origin',(0.,0.8,5.3));
#11998=CARTESIAN_POINT('Origin',(0.,0.8,5.8));
#11999=CARTESIAN_POINT('',(-0.685,0.8,5.8));
#12000=CARTESIAN_POINT('Origin',(0.,0.8,5.8));
#12001=CARTESIAN_POINT('',(-0.685,0.8,7.));
#12002=CARTESIAN_POINT('',(-0.685,0.8,5.8));
#12003=CARTESIAN_POINT('Origin',(0.,0.8,7.));
#12004=CARTESIAN_POINT('Origin',(0.,0.8,5.8));
#12005=CARTESIAN_POINT('Origin',(2.,-0.1,2.5));
#12006=CARTESIAN_POINT('',(1.725,0.,2.5));
#12007=CARTESIAN_POINT('Origin',(2.,0.,2.5));
#12008=CARTESIAN_POINT('',(1.725,1.7,2.5));
#12009=CARTESIAN_POINT('',(1.725,-0.1,2.5));
#12010=CARTESIAN_POINT('Origin',(2.,1.7,2.5));
#12011=CARTESIAN_POINT('Origin',(-2.,-0.1,6.5));
#12012=CARTESIAN_POINT('',(-2.275,0.,6.5));
#12013=CARTESIAN_POINT('Origin',(-2.,0.,6.5));
#12014=CARTESIAN_POINT('',(-2.275,1.7,6.5));
#12015=CARTESIAN_POINT('',(-2.275,-0.1,6.5));
#12016=CARTESIAN_POINT('Origin',(-2.,1.7,6.5));
#12017=CARTESIAN_POINT('Origin',(-2.,-0.1,2.5));
#12018=CARTESIAN_POINT('',(-2.275,0.,2.5));
#12019=CARTESIAN_POINT('Origin',(-2.,0.,2.5));
#12020=CARTESIAN_POINT('',(-2.275,1.7,2.5));
#12021=CARTESIAN_POINT('',(-2.275,-0.1,2.5));
#12022=CARTESIAN_POINT('Origin',(-2.,1.7,2.5));
#12023=CARTESIAN_POINT('Origin',(2.,-0.1,6.5));
#12024=CARTESIAN_POINT('',(1.725,0.,6.5));
#12025=CARTESIAN_POINT('Origin',(2.,0.,6.5));
#12026=CARTESIAN_POINT('',(1.725,1.7,6.5));
#12027=CARTESIAN_POINT('',(1.725,-0.1,6.5));
#12028=CARTESIAN_POINT('Origin',(2.,1.7,6.5));
#12029=CARTESIAN_POINT('Origin',(0.,-0.1,4.5));
#12030=CARTESIAN_POINT('',(-0.6,0.,4.5));
#12031=CARTESIAN_POINT('Origin',(0.,0.,4.5));
#12032=CARTESIAN_POINT('',(-0.6,1.2,4.5));
#12033=CARTESIAN_POINT('',(-0.6,-0.1,4.5));
#12034=CARTESIAN_POINT('Origin',(0.,1.2,4.5));
#12035=CARTESIAN_POINT('Origin',(0.,1.2,4.5));
#12036=CARTESIAN_POINT('Origin',(2.5,1.7,2.));
#12037=CARTESIAN_POINT('',(2.5,1.7,2.));
#12038=CARTESIAN_POINT('',(-2.5,1.7,2.));
#12039=CARTESIAN_POINT('',(2.5,1.7,2.));
#12040=CARTESIAN_POINT('',(-2.5,1.7,7.));
#12041=CARTESIAN_POINT('',(-2.5,1.7,2.));
#12042=CARTESIAN_POINT('',(2.5,1.7,7.));
#12043=CARTESIAN_POINT('',(2.5,1.7,7.));
#12044=CARTESIAN_POINT('',(2.5,1.7,2.));
#12045=CARTESIAN_POINT('Origin',(2.5,0.,2.));
#12046=CARTESIAN_POINT('',(2.5,0.,2.));
#12047=CARTESIAN_POINT('',(2.5,0.,2.));
#12048=CARTESIAN_POINT('',(2.5,0.,7.));
#12049=CARTESIAN_POINT('',(2.5,0.,7.));
#12050=CARTESIAN_POINT('',(2.5,0.,2.));
#12051=CARTESIAN_POINT('Origin',(-2.5,0.,2.));
#12052=CARTESIAN_POINT('',(-2.5,0.,2.));
#12053=CARTESIAN_POINT('',(-2.5,0.,2.));
#12054=CARTESIAN_POINT('',(-2.5,0.,7.));
#12055=CARTESIAN_POINT('',(-2.5,0.,7.));
#12056=CARTESIAN_POINT('',(-2.5,0.,2.));
#12057=CARTESIAN_POINT('Origin',(-2.5,1.7,2.));
#12058=CARTESIAN_POINT('',(-2.5,1.7,2.));
#12059=CARTESIAN_POINT('',(-2.5,1.7,7.));
#12060=CARTESIAN_POINT('Origin',(0.,0.85,7.));
#12061=CARTESIAN_POINT('Origin',(0.,0.85,2.));
#14299=UNCERTAINTY_MEASURE_WITH_UNIT(LENGTH_MEASURE(0.001),#14393,
'DISTANCE_ACCURACY_VALUE',
'Maximum model space distance between geometric entities at asserted c
onnectivities');
#14344=UNCERTAINTY_MEASURE_WITH_UNIT(LENGTH_MEASURE(0.001),#14393,
'DISTANCE_ACCURACY_VALUE',
'Maximum model space distance between geometric entities at asserted c
onnectivities');
#14347=(
GEOMETRIC_REPRESENTATION_CONTEXT(3)
GLOBAL_UNCERTAINTY_ASSIGNED_CONTEXT((#14299))
GLOBAL_UNIT_ASSIGNED_CONTEXT((#14393,#14395,#14396))
REPRESENTATION_CONTEXT('','3D')
);
#14392=(
GEOMETRIC_REPRESENTATION_CONTEXT(3)
GLOBAL_UNCERTAINTY_ASSIGNED_CONTEXT((#14344))
GLOBAL_UNIT_ASSIGNED_CONTEXT((#14393,#14395,#14396))
REPRESENTATION_CONTEXT('','3D')
);
#14393=(
LENGTH_UNIT()
NAMED_UNIT(*)
SI_UNIT(.CENTI.,.METRE.)
);
#14395=(
NAMED_UNIT(*)
PLANE_ANGLE_UNIT()
SI_UNIT($,.RADIAN.)
);
#14396=(
NAMED_UNIT(*)
SI_UNIT($,.STERADIAN.)
SOLID_ANGLE_UNIT()
);
#14399=SHAPE_DEFINITION_REPRESENTATION(#14446,#14585);
#14446=PRODUCT_DEFINITION_SHAPE('',$,#14633);
#14585=SHAPE_REPRESENTATION('',(#8386),#14347);
#14630=PRODUCT_DEFINITION_CONTEXT('part definition',#14773,'design');
#14633=PRODUCT_DEFINITION('Front cylinder cap','Front cylinder cap',#14680,
#14630);
#14680=PRODUCT_DEFINITION_FORMATION('',$,#14777);
#14773=APPLICATION_CONTEXT(
'Core Data for Automotive Mechanical Design Process');
#14774=PRODUCT_CONTEXT('part definition',#14773,'mechanical');
#14777=PRODUCT('Front cylinder cap','Front cylinder cap',
'Front cylinder cap',(#14774));
#14871=COLOUR_RGB('Light Blue',0.38,0.62,0.78);
#14872=FILL_AREA_STYLE_COLOUR('',#14871);
#14873=FILL_AREA_STYLE('',(#14872));
#14874=SURFACE_STYLE_FILL_AREA(#14873);
#14875=SURFACE_SIDE_STYLE('',(#14874));
#14876=SURFACE_STYLE_USAGE(.BOTH.,#14875);
#14877=PRESENTATION_STYLE_ASSIGNMENT((#14876));
ENDSEC;
END-ISO-10303-21;
